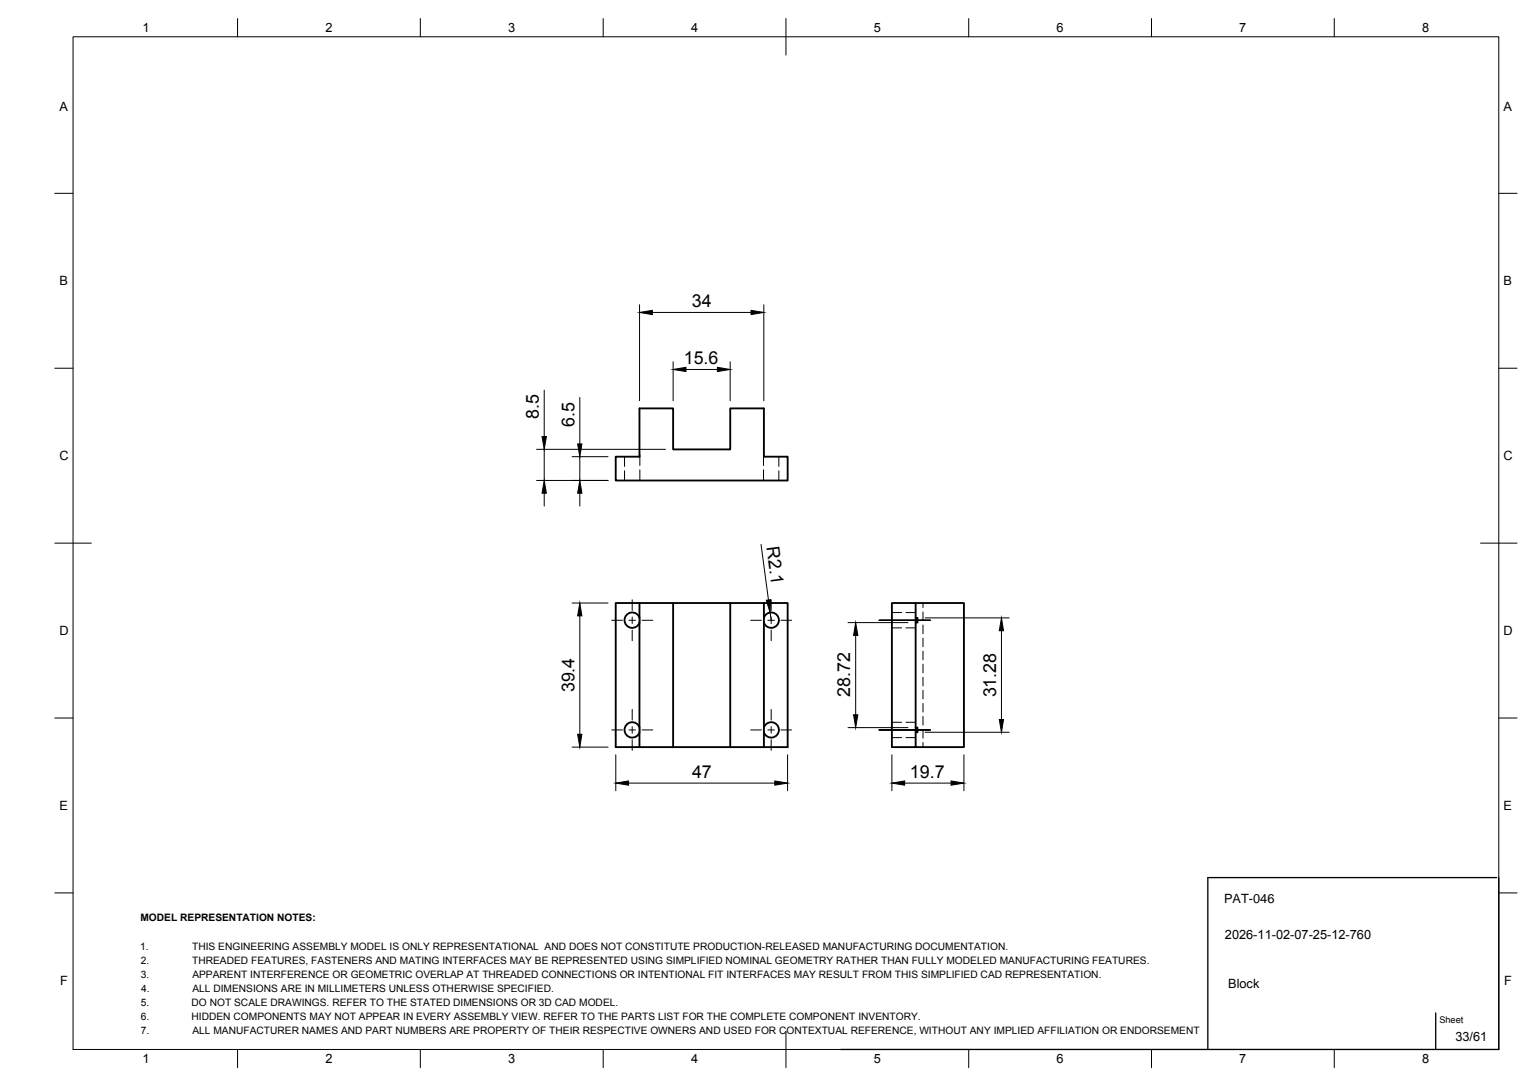
ISO-10303-21;
HEADER;
/* Generated by software containing ST-Developer
 * from STEP Tools, Inc. (www.steptools.com) 
 */

FILE_DESCRIPTION(
/* description */ ('Gear mesh backlash fixture'),
/* implementation_level */ '2;1');

FILE_NAME(
/* name */ 'Block.step',
/* time_stamp */ '2026-10-28T03:26:00-07:00',
/* author */ (''),
/* organization */ (''),
/* preprocessor_version */ 'ST-DEVELOPER v20.2',
/* originating_system */ 'Autodesk Translation Framework v15.17.0.0',
/* authorisation */ '');

FILE_SCHEMA (('AUTOMOTIVE_DESIGN { 1 0 10303 214 3 1 1 }'));
ENDSEC;

DATA;
#10=MECHANICAL_DESIGN_GEOMETRIC_PRESENTATION_REPRESENTATION('',(#1046),#57900);
#939=SHAPE_REPRESENTATION_RELATIONSHIP('SRR','None',#58137,#989);
#989=ADVANCED_BREP_SHAPE_REPRESENTATION('',(#1110),#57870);
#1046=STYLED_ITEM('',(#58444),#1110);
#1110=MANIFOLD_SOLID_BREP('Body1',#13607);
#1276=FACE_BOUND('',#2886,.T.);
#1277=FACE_BOUND('',#2887,.T.);
#1278=FACE_BOUND('',#2888,.T.);
#1279=FACE_BOUND('',#2889,.T.);
#1474=PLANE('',#14803);
#1475=PLANE('',#14809);
#1476=PLANE('',#14815);
#1477=PLANE('',#14821);
#1478=PLANE('',#14827);
#1479=PLANE('',#14828);
#1480=PLANE('',#14829);
#1481=PLANE('',#14830);
#1482=PLANE('',#14831);
#1483=PLANE('',#14832);
#1484=PLANE('',#14833);
#1485=PLANE('',#14834);
#1486=PLANE('',#14835);
#1487=PLANE('',#14836);
#1488=PLANE('',#14837);
#1489=PLANE('',#14838);
#1490=PLANE('',#14839);
#1491=PLANE('',#14840);
#1974=FACE_OUTER_BOUND('',#2872,.T.);
#1975=FACE_OUTER_BOUND('',#2873,.T.);
#1976=FACE_OUTER_BOUND('',#2874,.T.);
#1977=FACE_OUTER_BOUND('',#2875,.T.);
#1978=FACE_OUTER_BOUND('',#2876,.T.);
#1979=FACE_OUTER_BOUND('',#2877,.T.);
#1980=FACE_OUTER_BOUND('',#2878,.T.);
#1981=FACE_OUTER_BOUND('',#2879,.T.);
#1982=FACE_OUTER_BOUND('',#2880,.T.);
#1983=FACE_OUTER_BOUND('',#2881,.T.);
#1984=FACE_OUTER_BOUND('',#2882,.T.);
#1985=FACE_OUTER_BOUND('',#2883,.T.);
#1986=FACE_OUTER_BOUND('',#2884,.T.);
#1987=FACE_OUTER_BOUND('',#2885,.T.);
#1988=FACE_OUTER_BOUND('',#2890,.T.);
#1989=FACE_OUTER_BOUND('',#2891,.T.);
#1990=FACE_OUTER_BOUND('',#2892,.T.);
#1991=FACE_OUTER_BOUND('',#2893,.T.);
#1992=FACE_OUTER_BOUND('',#2894,.T.);
#1993=FACE_OUTER_BOUND('',#2895,.T.);
#1994=FACE_OUTER_BOUND('',#2896,.T.);
#1995=FACE_OUTER_BOUND('',#2897,.T.);
#2872=EDGE_LOOP('',(#10125,#10126));
#2873=EDGE_LOOP('',(#10127,#10128,#10129,#10130,#10131,#10132,#10133,#10134));
#2874=EDGE_LOOP('',(#10135,#10136));
#2875=EDGE_LOOP('',(#10137,#10138,#10139,#10140,#10141,#10142,#10143,#10144));
#2876=EDGE_LOOP('',(#10145,#10146));
#2877=EDGE_LOOP('',(#10147,#10148,#10149,#10150,#10151,#10152,#10153,#10154));
#2878=EDGE_LOOP('',(#10155,#10156));
#2879=EDGE_LOOP('',(#10157,#10158,#10159,#10160,#10161,#10162,#10163,#10164));
#2880=EDGE_LOOP('',(#10165,#10166,#10167,#10168,#10169,#10170,#10171,#10172,
#10173,#10174,#10175,#10176));
#2881=EDGE_LOOP('',(#10177,#10178,#10179,#10180,#10181,#10182,#10183,#10184,
#10185,#10186,#10187,#10188));
#2882=EDGE_LOOP('',(#10189,#10190,#10191,#10192,#10193,#10194,#10195,#10196,
#10197,#10198,#10199,#10200));
#2883=EDGE_LOOP('',(#10201,#10202,#10203,#10204,#10205,#10206,#10207,#10208,
#10209,#10210));
#2884=EDGE_LOOP('',(#10211,#10212,#10213,#10214));
#2885=EDGE_LOOP('',(#10215,#10216,#10217,#10218));
#2886=EDGE_LOOP('',(#10219));
#2887=EDGE_LOOP('',(#10220));
#2888=EDGE_LOOP('',(#10221));
#2889=EDGE_LOOP('',(#10222));
#2890=EDGE_LOOP('',(#10223,#10224,#10225,#10226));
#2891=EDGE_LOOP('',(#10227,#10228,#10229,#10230,#10231,#10232,#10233,#10234,
#10235,#10236));
#2892=EDGE_LOOP('',(#10237,#10238,#10239,#10240));
#2893=EDGE_LOOP('',(#10241,#10242,#10243,#10244));
#2894=EDGE_LOOP('',(#10245,#10246,#10247,#10248));
#2895=EDGE_LOOP('',(#10249,#10250,#10251,#10252));
#2896=EDGE_LOOP('',(#10253,#10254,#10255,#10256));
#2897=EDGE_LOOP('',(#10257,#10258,#10259,#10260,#10261,#10262,#10263,#10264,
#10265,#10266,#10267,#10268));
#3715=LINE('',#21048,#4604);
#3716=LINE('',#21052,#4605);
#3717=LINE('',#21056,#4606);
#3718=LINE('',#21060,#4607);
#3719=LINE('',#21064,#4608);
#3720=LINE('',#21068,#4609);
#3721=LINE('',#21072,#4610);
#3722=LINE('',#21076,#4611);
#3723=LINE('',#21080,#4612);
#3724=LINE('',#21084,#4613);
#3725=LINE('',#21088,#4614);
#3726=LINE('',#21092,#4615);
#3727=LINE('',#21096,#4616);
#3728=LINE('',#21100,#4617);
#3729=LINE('',#21104,#4618);
#3730=LINE('',#21108,#4619);
#3731=LINE('',#21110,#4620);
#3732=LINE('',#21112,#4621);
#3733=LINE('',#21114,#4622);
#3734=LINE('',#21116,#4623);
#3735=LINE('',#21118,#4624);
#3736=LINE('',#21119,#4625);
#3737=LINE('',#21121,#4626);
#3738=LINE('',#21123,#4627);
#3739=LINE('',#21125,#4628);
#3740=LINE('',#21127,#4629);
#3741=LINE('',#21129,#4630);
#3742=LINE('',#21130,#4631);
#3743=LINE('',#21133,#4632);
#3744=LINE('',#21135,#4633);
#3745=LINE('',#21137,#4634);
#3746=LINE('',#21139,#4635);
#3747=LINE('',#21140,#4636);
#3748=LINE('',#21142,#4637);
#3749=LINE('',#21144,#4638);
#3750=LINE('',#21146,#4639);
#3751=LINE('',#21148,#4640);
#3752=LINE('',#21149,#4641);
#3753=LINE('',#21152,#4642);
#3754=LINE('',#21153,#4643);
#3755=LINE('',#21156,#4644);
#3756=LINE('',#21157,#4645);
#3757=LINE('',#21160,#4646);
#3758=LINE('',#21161,#4647);
#3759=LINE('',#21164,#4648);
#3760=LINE('',#21165,#4649);
#3761=LINE('',#21167,#4650);
#3762=LINE('',#21170,#4651);
#3763=LINE('',#21171,#4652);
#3764=LINE('',#21174,#4653);
#3765=LINE('',#21175,#4654);
#3766=LINE('',#21178,#4655);
#3767=LINE('',#21179,#4656);
#3768=LINE('',#21182,#4657);
#3769=LINE('',#21183,#4658);
#3770=LINE('',#21185,#4659);
#4604=VECTOR('',#17100,1.);
#4605=VECTOR('',#17105,1.);
#4606=VECTOR('',#17108,0.21);
#4607=VECTOR('',#17113,1.);
#4608=VECTOR('',#17116,1.);
#4609=VECTOR('',#17121,1.);
#4610=VECTOR('',#17124,0.21);
#4611=VECTOR('',#17129,1.);
#4612=VECTOR('',#17132,1.);
#4613=VECTOR('',#17137,1.);
#4614=VECTOR('',#17140,0.21);
#4615=VECTOR('',#17145,1.);
#4616=VECTOR('',#17148,1.);
#4617=VECTOR('',#17153,1.);
#4618=VECTOR('',#17156,0.21);
#4619=VECTOR('',#17161,1.);
#4620=VECTOR('',#17164,1.);
#4621=VECTOR('',#17165,1.);
#4622=VECTOR('',#17166,1.);
#4623=VECTOR('',#17167,1.);
#4624=VECTOR('',#17168,1.);
#4625=VECTOR('',#17169,1.);
#4626=VECTOR('',#17172,1.);
#4627=VECTOR('',#17173,1.);
#4628=VECTOR('',#17174,1.);
#4629=VECTOR('',#17175,1.);
#4630=VECTOR('',#17176,1.);
#4631=VECTOR('',#17177,1.);
#4632=VECTOR('',#17180,1.);
#4633=VECTOR('',#17181,1.);
#4634=VECTOR('',#17182,1.);
#4635=VECTOR('',#17183,1.);
#4636=VECTOR('',#17184,1.);
#4637=VECTOR('',#17185,1.);
#4638=VECTOR('',#17186,1.);
#4639=VECTOR('',#17187,1.);
#4640=VECTOR('',#17188,1.);
#4641=VECTOR('',#17189,1.);
#4642=VECTOR('',#17192,1.);
#4643=VECTOR('',#17193,1.);
#4644=VECTOR('',#17196,1.);
#4645=VECTOR('',#17197,1.);
#4646=VECTOR('',#17200,1.);
#4647=VECTOR('',#17201,1.);
#4648=VECTOR('',#17204,1.);
#4649=VECTOR('',#17205,1.);
#4650=VECTOR('',#17208,1.);
#4651=VECTOR('',#17211,1.);
#4652=VECTOR('',#17212,1.);
#4653=VECTOR('',#17215,1.);
#4654=VECTOR('',#17216,1.);
#4655=VECTOR('',#17219,1.);
#4656=VECTOR('',#17220,1.);
#4657=VECTOR('',#17223,1.);
#4658=VECTOR('',#17224,1.);
#4659=VECTOR('',#17227,1.);
#5483=CIRCLE('',#14804,0.21);
#5484=CIRCLE('',#14806,0.21);
#5485=CIRCLE('',#14807,0.21);
#5486=CIRCLE('',#14808,0.21);
#5487=CIRCLE('',#14810,0.21);
#5488=CIRCLE('',#14812,0.21);
#5489=CIRCLE('',#14813,0.21);
#5490=CIRCLE('',#14814,0.21);
#5491=CIRCLE('',#14816,0.21);
#5492=CIRCLE('',#14818,0.21);
#5493=CIRCLE('',#14819,0.21);
#5494=CIRCLE('',#14820,0.21);
#5495=CIRCLE('',#14822,0.21);
#5496=CIRCLE('',#14824,0.21);
#5497=CIRCLE('',#14825,0.21);
#5498=CIRCLE('',#14826,0.21);
#6199=VERTEX_POINT('',#21046);
#6200=VERTEX_POINT('',#21047);
#6201=VERTEX_POINT('',#21051);
#6202=VERTEX_POINT('',#21053);
#6203=VERTEX_POINT('',#21055);
#6204=VERTEX_POINT('',#21058);
#6205=VERTEX_POINT('',#21062);
#6206=VERTEX_POINT('',#21063);
#6207=VERTEX_POINT('',#21067);
#6208=VERTEX_POINT('',#21069);
#6209=VERTEX_POINT('',#21071);
#6210=VERTEX_POINT('',#21074);
#6211=VERTEX_POINT('',#21078);
#6212=VERTEX_POINT('',#21079);
#6213=VERTEX_POINT('',#21083);
#6214=VERTEX_POINT('',#21085);
#6215=VERTEX_POINT('',#21087);
#6216=VERTEX_POINT('',#21090);
#6217=VERTEX_POINT('',#21094);
#6218=VERTEX_POINT('',#21095);
#6219=VERTEX_POINT('',#21099);
#6220=VERTEX_POINT('',#21101);
#6221=VERTEX_POINT('',#21103);
#6222=VERTEX_POINT('',#21106);
#6223=VERTEX_POINT('',#21111);
#6224=VERTEX_POINT('',#21113);
#6225=VERTEX_POINT('',#21115);
#6226=VERTEX_POINT('',#21117);
#6227=VERTEX_POINT('',#21122);
#6228=VERTEX_POINT('',#21124);
#6229=VERTEX_POINT('',#21126);
#6230=VERTEX_POINT('',#21128);
#6231=VERTEX_POINT('',#21132);
#6232=VERTEX_POINT('',#21134);
#6233=VERTEX_POINT('',#21136);
#6234=VERTEX_POINT('',#21138);
#6235=VERTEX_POINT('',#21141);
#6236=VERTEX_POINT('',#21143);
#6237=VERTEX_POINT('',#21145);
#6238=VERTEX_POINT('',#21147);
#6239=VERTEX_POINT('',#21151);
#6240=VERTEX_POINT('',#21155);
#6241=VERTEX_POINT('',#21159);
#6242=VERTEX_POINT('',#21163);
#6243=VERTEX_POINT('',#21169);
#6244=VERTEX_POINT('',#21173);
#6245=VERTEX_POINT('',#21177);
#6246=VERTEX_POINT('',#21181);
#7649=EDGE_CURVE('',#6199,#6200,#3715,.T.);
#7650=EDGE_CURVE('',#6199,#6200,#5483,.T.);
#7651=EDGE_CURVE('',#6201,#6199,#3716,.T.);
#7652=EDGE_CURVE('',#6202,#6201,#5484,.T.);
#7653=EDGE_CURVE('',#6202,#6203,#3717,.T.);
#7654=EDGE_CURVE('',#6203,#6203,#5485,.T.);
#7655=EDGE_CURVE('',#6204,#6202,#5486,.T.);
#7656=EDGE_CURVE('',#6200,#6204,#3718,.T.);
#7657=EDGE_CURVE('',#6205,#6206,#3719,.T.);
#7658=EDGE_CURVE('',#6205,#6206,#5487,.T.);
#7659=EDGE_CURVE('',#6207,#6205,#3720,.T.);
#7660=EDGE_CURVE('',#6208,#6207,#5488,.T.);
#7661=EDGE_CURVE('',#6208,#6209,#3721,.T.);
#7662=EDGE_CURVE('',#6209,#6209,#5489,.T.);
#7663=EDGE_CURVE('',#6210,#6208,#5490,.T.);
#7664=EDGE_CURVE('',#6206,#6210,#3722,.T.);
#7665=EDGE_CURVE('',#6211,#6212,#3723,.T.);
#7666=EDGE_CURVE('',#6211,#6212,#5491,.T.);
#7667=EDGE_CURVE('',#6213,#6211,#3724,.T.);
#7668=EDGE_CURVE('',#6214,#6213,#5492,.T.);
#7669=EDGE_CURVE('',#6214,#6215,#3725,.T.);
#7670=EDGE_CURVE('',#6215,#6215,#5493,.T.);
#7671=EDGE_CURVE('',#6216,#6214,#5494,.T.);
#7672=EDGE_CURVE('',#6212,#6216,#3726,.T.);
#7673=EDGE_CURVE('',#6217,#6218,#3727,.T.);
#7674=EDGE_CURVE('',#6217,#6218,#5495,.T.);
#7675=EDGE_CURVE('',#6219,#6217,#3728,.T.);
#7676=EDGE_CURVE('',#6220,#6219,#5496,.T.);
#7677=EDGE_CURVE('',#6220,#6221,#3729,.T.);
#7678=EDGE_CURVE('',#6221,#6221,#5497,.T.);
#7679=EDGE_CURVE('',#6222,#6220,#5498,.T.);
#7680=EDGE_CURVE('',#6218,#6222,#3730,.T.);
#7681=EDGE_CURVE('',#6204,#6213,#3731,.T.);
#7682=EDGE_CURVE('',#6216,#6223,#3732,.T.);
#7683=EDGE_CURVE('',#6224,#6223,#3733,.T.);
#7684=EDGE_CURVE('',#6224,#6225,#3734,.T.);
#7685=EDGE_CURVE('',#6226,#6225,#3735,.T.);
#7686=EDGE_CURVE('',#6226,#6201,#3736,.T.);
#7687=EDGE_CURVE('',#6210,#6219,#3737,.T.);
#7688=EDGE_CURVE('',#6222,#6227,#3738,.T.);
#7689=EDGE_CURVE('',#6228,#6227,#3739,.T.);
#7690=EDGE_CURVE('',#6229,#6228,#3740,.T.);
#7691=EDGE_CURVE('',#6230,#6229,#3741,.T.);
#7692=EDGE_CURVE('',#6230,#6207,#3742,.T.);
#7693=EDGE_CURVE('',#6223,#6231,#3743,.T.);
#7694=EDGE_CURVE('',#6231,#6232,#3744,.T.);
#7695=EDGE_CURVE('',#6232,#6233,#3745,.T.);
#7696=EDGE_CURVE('',#6233,#6234,#3746,.T.);
#7697=EDGE_CURVE('',#6234,#6230,#3747,.T.);
#7698=EDGE_CURVE('',#6229,#6235,#3748,.T.);
#7699=EDGE_CURVE('',#6235,#6236,#3749,.T.);
#7700=EDGE_CURVE('',#6236,#6237,#3750,.T.);
#7701=EDGE_CURVE('',#6237,#6238,#3751,.T.);
#7702=EDGE_CURVE('',#6238,#6224,#3752,.T.);
#7703=EDGE_CURVE('',#6239,#6226,#3753,.T.);
#7704=EDGE_CURVE('',#6231,#6239,#3754,.T.);
#7705=EDGE_CURVE('',#6240,#6239,#3755,.T.);
#7706=EDGE_CURVE('',#6232,#6240,#3756,.T.);
#7707=EDGE_CURVE('',#6241,#6240,#3757,.T.);
#7708=EDGE_CURVE('',#6233,#6241,#3758,.T.);
#7709=EDGE_CURVE('',#6242,#6241,#3759,.T.);
#7710=EDGE_CURVE('',#6234,#6242,#3760,.T.);
#7711=EDGE_CURVE('',#6227,#6242,#3761,.T.);
#7712=EDGE_CURVE('',#6243,#6228,#3762,.T.);
#7713=EDGE_CURVE('',#6235,#6243,#3763,.T.);
#7714=EDGE_CURVE('',#6244,#6243,#3764,.T.);
#7715=EDGE_CURVE('',#6236,#6244,#3765,.T.);
#7716=EDGE_CURVE('',#6245,#6244,#3766,.T.);
#7717=EDGE_CURVE('',#6237,#6245,#3767,.T.);
#7718=EDGE_CURVE('',#6246,#6245,#3768,.T.);
#7719=EDGE_CURVE('',#6238,#6246,#3769,.T.);
#7720=EDGE_CURVE('',#6225,#6246,#3770,.T.);
#10125=ORIENTED_EDGE('',*,*,#7649,.F.);
#10126=ORIENTED_EDGE('',*,*,#7650,.T.);
#10127=ORIENTED_EDGE('',*,*,#7651,.F.);
#10128=ORIENTED_EDGE('',*,*,#7652,.F.);
#10129=ORIENTED_EDGE('',*,*,#7653,.T.);
#10130=ORIENTED_EDGE('',*,*,#7654,.F.);
#10131=ORIENTED_EDGE('',*,*,#7653,.F.);
#10132=ORIENTED_EDGE('',*,*,#7655,.F.);
#10133=ORIENTED_EDGE('',*,*,#7656,.F.);
#10134=ORIENTED_EDGE('',*,*,#7650,.F.);
#10135=ORIENTED_EDGE('',*,*,#7657,.F.);
#10136=ORIENTED_EDGE('',*,*,#7658,.T.);
#10137=ORIENTED_EDGE('',*,*,#7659,.F.);
#10138=ORIENTED_EDGE('',*,*,#7660,.F.);
#10139=ORIENTED_EDGE('',*,*,#7661,.T.);
#10140=ORIENTED_EDGE('',*,*,#7662,.F.);
#10141=ORIENTED_EDGE('',*,*,#7661,.F.);
#10142=ORIENTED_EDGE('',*,*,#7663,.F.);
#10143=ORIENTED_EDGE('',*,*,#7664,.F.);
#10144=ORIENTED_EDGE('',*,*,#7658,.F.);
#10145=ORIENTED_EDGE('',*,*,#7665,.F.);
#10146=ORIENTED_EDGE('',*,*,#7666,.T.);
#10147=ORIENTED_EDGE('',*,*,#7667,.F.);
#10148=ORIENTED_EDGE('',*,*,#7668,.F.);
#10149=ORIENTED_EDGE('',*,*,#7669,.T.);
#10150=ORIENTED_EDGE('',*,*,#7670,.F.);
#10151=ORIENTED_EDGE('',*,*,#7669,.F.);
#10152=ORIENTED_EDGE('',*,*,#7671,.F.);
#10153=ORIENTED_EDGE('',*,*,#7672,.F.);
#10154=ORIENTED_EDGE('',*,*,#7666,.F.);
#10155=ORIENTED_EDGE('',*,*,#7673,.F.);
#10156=ORIENTED_EDGE('',*,*,#7674,.T.);
#10157=ORIENTED_EDGE('',*,*,#7675,.F.);
#10158=ORIENTED_EDGE('',*,*,#7676,.F.);
#10159=ORIENTED_EDGE('',*,*,#7677,.T.);
#10160=ORIENTED_EDGE('',*,*,#7678,.F.);
#10161=ORIENTED_EDGE('',*,*,#7677,.F.);
#10162=ORIENTED_EDGE('',*,*,#7679,.F.);
#10163=ORIENTED_EDGE('',*,*,#7680,.F.);
#10164=ORIENTED_EDGE('',*,*,#7674,.F.);
#10165=ORIENTED_EDGE('',*,*,#7651,.T.);
#10166=ORIENTED_EDGE('',*,*,#7649,.T.);
#10167=ORIENTED_EDGE('',*,*,#7656,.T.);
#10168=ORIENTED_EDGE('',*,*,#7681,.T.);
#10169=ORIENTED_EDGE('',*,*,#7667,.T.);
#10170=ORIENTED_EDGE('',*,*,#7665,.T.);
#10171=ORIENTED_EDGE('',*,*,#7672,.T.);
#10172=ORIENTED_EDGE('',*,*,#7682,.T.);
#10173=ORIENTED_EDGE('',*,*,#7683,.F.);
#10174=ORIENTED_EDGE('',*,*,#7684,.T.);
#10175=ORIENTED_EDGE('',*,*,#7685,.F.);
#10176=ORIENTED_EDGE('',*,*,#7686,.T.);
#10177=ORIENTED_EDGE('',*,*,#7659,.T.);
#10178=ORIENTED_EDGE('',*,*,#7657,.T.);
#10179=ORIENTED_EDGE('',*,*,#7664,.T.);
#10180=ORIENTED_EDGE('',*,*,#7687,.T.);
#10181=ORIENTED_EDGE('',*,*,#7675,.T.);
#10182=ORIENTED_EDGE('',*,*,#7673,.T.);
#10183=ORIENTED_EDGE('',*,*,#7680,.T.);
#10184=ORIENTED_EDGE('',*,*,#7688,.T.);
#10185=ORIENTED_EDGE('',*,*,#7689,.F.);
#10186=ORIENTED_EDGE('',*,*,#7690,.F.);
#10187=ORIENTED_EDGE('',*,*,#7691,.F.);
#10188=ORIENTED_EDGE('',*,*,#7692,.T.);
#10189=ORIENTED_EDGE('',*,*,#7683,.T.);
#10190=ORIENTED_EDGE('',*,*,#7693,.T.);
#10191=ORIENTED_EDGE('',*,*,#7694,.T.);
#10192=ORIENTED_EDGE('',*,*,#7695,.T.);
#10193=ORIENTED_EDGE('',*,*,#7696,.T.);
#10194=ORIENTED_EDGE('',*,*,#7697,.T.);
#10195=ORIENTED_EDGE('',*,*,#7691,.T.);
#10196=ORIENTED_EDGE('',*,*,#7698,.T.);
#10197=ORIENTED_EDGE('',*,*,#7699,.T.);
#10198=ORIENTED_EDGE('',*,*,#7700,.T.);
#10199=ORIENTED_EDGE('',*,*,#7701,.T.);
#10200=ORIENTED_EDGE('',*,*,#7702,.T.);
#10201=ORIENTED_EDGE('',*,*,#7655,.T.);
#10202=ORIENTED_EDGE('',*,*,#7652,.T.);
#10203=ORIENTED_EDGE('',*,*,#7686,.F.);
#10204=ORIENTED_EDGE('',*,*,#7703,.F.);
#10205=ORIENTED_EDGE('',*,*,#7704,.F.);
#10206=ORIENTED_EDGE('',*,*,#7693,.F.);
#10207=ORIENTED_EDGE('',*,*,#7682,.F.);
#10208=ORIENTED_EDGE('',*,*,#7671,.T.);
#10209=ORIENTED_EDGE('',*,*,#7668,.T.);
#10210=ORIENTED_EDGE('',*,*,#7681,.F.);
#10211=ORIENTED_EDGE('',*,*,#7704,.T.);
#10212=ORIENTED_EDGE('',*,*,#7705,.F.);
#10213=ORIENTED_EDGE('',*,*,#7706,.F.);
#10214=ORIENTED_EDGE('',*,*,#7694,.F.);
#10215=ORIENTED_EDGE('',*,*,#7706,.T.);
#10216=ORIENTED_EDGE('',*,*,#7707,.F.);
#10217=ORIENTED_EDGE('',*,*,#7708,.F.);
#10218=ORIENTED_EDGE('',*,*,#7695,.F.);
#10219=ORIENTED_EDGE('',*,*,#7654,.T.);
#10220=ORIENTED_EDGE('',*,*,#7662,.T.);
#10221=ORIENTED_EDGE('',*,*,#7670,.T.);
#10222=ORIENTED_EDGE('',*,*,#7678,.T.);
#10223=ORIENTED_EDGE('',*,*,#7708,.T.);
#10224=ORIENTED_EDGE('',*,*,#7709,.F.);
#10225=ORIENTED_EDGE('',*,*,#7710,.F.);
#10226=ORIENTED_EDGE('',*,*,#7696,.F.);
#10227=ORIENTED_EDGE('',*,*,#7663,.T.);
#10228=ORIENTED_EDGE('',*,*,#7660,.T.);
#10229=ORIENTED_EDGE('',*,*,#7692,.F.);
#10230=ORIENTED_EDGE('',*,*,#7697,.F.);
#10231=ORIENTED_EDGE('',*,*,#7710,.T.);
#10232=ORIENTED_EDGE('',*,*,#7711,.F.);
#10233=ORIENTED_EDGE('',*,*,#7688,.F.);
#10234=ORIENTED_EDGE('',*,*,#7679,.T.);
#10235=ORIENTED_EDGE('',*,*,#7676,.T.);
#10236=ORIENTED_EDGE('',*,*,#7687,.F.);
#10237=ORIENTED_EDGE('',*,*,#7690,.T.);
#10238=ORIENTED_EDGE('',*,*,#7712,.F.);
#10239=ORIENTED_EDGE('',*,*,#7713,.F.);
#10240=ORIENTED_EDGE('',*,*,#7698,.F.);
#10241=ORIENTED_EDGE('',*,*,#7713,.T.);
#10242=ORIENTED_EDGE('',*,*,#7714,.F.);
#10243=ORIENTED_EDGE('',*,*,#7715,.F.);
#10244=ORIENTED_EDGE('',*,*,#7699,.F.);
#10245=ORIENTED_EDGE('',*,*,#7715,.T.);
#10246=ORIENTED_EDGE('',*,*,#7716,.F.);
#10247=ORIENTED_EDGE('',*,*,#7717,.F.);
#10248=ORIENTED_EDGE('',*,*,#7700,.F.);
#10249=ORIENTED_EDGE('',*,*,#7717,.T.);
#10250=ORIENTED_EDGE('',*,*,#7718,.F.);
#10251=ORIENTED_EDGE('',*,*,#7719,.F.);
#10252=ORIENTED_EDGE('',*,*,#7701,.F.);
#10253=ORIENTED_EDGE('',*,*,#7719,.T.);
#10254=ORIENTED_EDGE('',*,*,#7720,.F.);
#10255=ORIENTED_EDGE('',*,*,#7684,.F.);
#10256=ORIENTED_EDGE('',*,*,#7702,.F.);
#10257=ORIENTED_EDGE('',*,*,#7685,.T.);
#10258=ORIENTED_EDGE('',*,*,#7720,.T.);
#10259=ORIENTED_EDGE('',*,*,#7718,.T.);
#10260=ORIENTED_EDGE('',*,*,#7716,.T.);
#10261=ORIENTED_EDGE('',*,*,#7714,.T.);
#10262=ORIENTED_EDGE('',*,*,#7712,.T.);
#10263=ORIENTED_EDGE('',*,*,#7689,.T.);
#10264=ORIENTED_EDGE('',*,*,#7711,.T.);
#10265=ORIENTED_EDGE('',*,*,#7709,.T.);
#10266=ORIENTED_EDGE('',*,*,#7707,.T.);
#10267=ORIENTED_EDGE('',*,*,#7705,.T.);
#10268=ORIENTED_EDGE('',*,*,#7703,.T.);
#12697=CYLINDRICAL_SURFACE('',#14805,0.21);
#12698=CYLINDRICAL_SURFACE('',#14811,0.21);
#12699=CYLINDRICAL_SURFACE('',#14817,0.21);
#12700=CYLINDRICAL_SURFACE('',#14823,0.21);
#13091=ADVANCED_FACE('',(#1974),#1474,.T.);
#13092=ADVANCED_FACE('',(#1975),#12697,.F.);
#13093=ADVANCED_FACE('',(#1976),#1475,.T.);
#13094=ADVANCED_FACE('',(#1977),#12698,.F.);
#13095=ADVANCED_FACE('',(#1978),#1476,.T.);
#13096=ADVANCED_FACE('',(#1979),#12699,.F.);
#13097=ADVANCED_FACE('',(#1980),#1477,.T.);
#13098=ADVANCED_FACE('',(#1981),#12700,.F.);
#13099=ADVANCED_FACE('',(#1982),#1478,.T.);
#13100=ADVANCED_FACE('',(#1983),#1479,.T.);
#13101=ADVANCED_FACE('',(#1984),#1480,.T.);
#13102=ADVANCED_FACE('',(#1985),#1481,.T.);
#13103=ADVANCED_FACE('',(#1986),#1482,.T.);
#13104=ADVANCED_FACE('',(#1987,#1276,#1277,#1278,#1279),#1483,.T.);
#13105=ADVANCED_FACE('',(#1988),#1484,.T.);
#13106=ADVANCED_FACE('',(#1989),#1485,.T.);
#13107=ADVANCED_FACE('',(#1990),#1486,.T.);
#13108=ADVANCED_FACE('',(#1991),#1487,.T.);
#13109=ADVANCED_FACE('',(#1992),#1488,.T.);
#13110=ADVANCED_FACE('',(#1993),#1489,.T.);
#13111=ADVANCED_FACE('',(#1994),#1490,.T.);
#13112=ADVANCED_FACE('',(#1995),#1491,.T.);
#13607=CLOSED_SHELL('',(#13091,#13092,#13093,#13094,#13095,#13096,#13097,
#13098,#13099,#13100,#13101,#13102,#13103,#13104,#13105,#13106,#13107,#13108,
#13109,#13110,#13111,#13112));
#14802=AXIS2_PLACEMENT_3D('',#21044,#17096,#17097);
#14803=AXIS2_PLACEMENT_3D('',#21045,#17098,#17099);
#14804=AXIS2_PLACEMENT_3D('',#21049,#17101,#17102);
#14805=AXIS2_PLACEMENT_3D('',#21050,#17103,#17104);
#14806=AXIS2_PLACEMENT_3D('',#21054,#17106,#17107);
#14807=AXIS2_PLACEMENT_3D('',#21057,#17109,#17110);
#14808=AXIS2_PLACEMENT_3D('',#21059,#17111,#17112);
#14809=AXIS2_PLACEMENT_3D('',#21061,#17114,#17115);
#14810=AXIS2_PLACEMENT_3D('',#21065,#17117,#17118);
#14811=AXIS2_PLACEMENT_3D('',#21066,#17119,#17120);
#14812=AXIS2_PLACEMENT_3D('',#21070,#17122,#17123);
#14813=AXIS2_PLACEMENT_3D('',#21073,#17125,#17126);
#14814=AXIS2_PLACEMENT_3D('',#21075,#17127,#17128);
#14815=AXIS2_PLACEMENT_3D('',#21077,#17130,#17131);
#14816=AXIS2_PLACEMENT_3D('',#21081,#17133,#17134);
#14817=AXIS2_PLACEMENT_3D('',#21082,#17135,#17136);
#14818=AXIS2_PLACEMENT_3D('',#21086,#17138,#17139);
#14819=AXIS2_PLACEMENT_3D('',#21089,#17141,#17142);
#14820=AXIS2_PLACEMENT_3D('',#21091,#17143,#17144);
#14821=AXIS2_PLACEMENT_3D('',#21093,#17146,#17147);
#14822=AXIS2_PLACEMENT_3D('',#21097,#17149,#17150);
#14823=AXIS2_PLACEMENT_3D('',#21098,#17151,#17152);
#14824=AXIS2_PLACEMENT_3D('',#21102,#17154,#17155);
#14825=AXIS2_PLACEMENT_3D('',#21105,#17157,#17158);
#14826=AXIS2_PLACEMENT_3D('',#21107,#17159,#17160);
#14827=AXIS2_PLACEMENT_3D('',#21109,#17162,#17163);
#14828=AXIS2_PLACEMENT_3D('',#21120,#17170,#17171);
#14829=AXIS2_PLACEMENT_3D('',#21131,#17178,#17179);
#14830=AXIS2_PLACEMENT_3D('',#21150,#17190,#17191);
#14831=AXIS2_PLACEMENT_3D('',#21154,#17194,#17195);
#14832=AXIS2_PLACEMENT_3D('',#21158,#17198,#17199);
#14833=AXIS2_PLACEMENT_3D('',#21162,#17202,#17203);
#14834=AXIS2_PLACEMENT_3D('',#21166,#17206,#17207);
#14835=AXIS2_PLACEMENT_3D('',#21168,#17209,#17210);
#14836=AXIS2_PLACEMENT_3D('',#21172,#17213,#17214);
#14837=AXIS2_PLACEMENT_3D('',#21176,#17217,#17218);
#14838=AXIS2_PLACEMENT_3D('',#21180,#17221,#17222);
#14839=AXIS2_PLACEMENT_3D('',#21184,#17225,#17226);
#14840=AXIS2_PLACEMENT_3D('',#21186,#17228,#17229);
#17096=DIRECTION('axis',(0.,0.,1.));
#17097=DIRECTION('refdir',(1.,0.,0.));
#17098=DIRECTION('center_axis',(0.,0.,1.));
#17099=DIRECTION('ref_axis',(1.,0.,0.));
#17100=DIRECTION('',(-1.,0.,0.));
#17101=DIRECTION('center_axis',(0.,0.,1.));
#17102=DIRECTION('ref_axis',(1.,0.,0.));
#17103=DIRECTION('center_axis',(0.,0.,1.));
#17104=DIRECTION('ref_axis',(1.,0.,0.));
#17105=DIRECTION('',(0.,0.,-1.));
#17106=DIRECTION('center_axis',(0.,0.,1.));
#17107=DIRECTION('ref_axis',(1.,0.,0.));
#17108=DIRECTION('',(0.,0.,1.));
#17109=DIRECTION('center_axis',(0.,0.,-1.));
#17110=DIRECTION('ref_axis',(1.,0.,0.));
#17111=DIRECTION('center_axis',(0.,0.,1.));
#17112=DIRECTION('ref_axis',(1.,0.,0.));
#17113=DIRECTION('',(0.,0.,1.));
#17114=DIRECTION('center_axis',(0.,0.,1.));
#17115=DIRECTION('ref_axis',(1.,0.,0.));
#17116=DIRECTION('',(1.,0.,0.));
#17117=DIRECTION('center_axis',(0.,0.,1.));
#17118=DIRECTION('ref_axis',(1.,0.,0.));
#17119=DIRECTION('center_axis',(0.,0.,1.));
#17120=DIRECTION('ref_axis',(1.,0.,0.));
#17121=DIRECTION('',(0.,0.,-1.));
#17122=DIRECTION('center_axis',(0.,0.,1.));
#17123=DIRECTION('ref_axis',(1.,0.,0.));
#17124=DIRECTION('',(0.,0.,1.));
#17125=DIRECTION('center_axis',(0.,0.,-1.));
#17126=DIRECTION('ref_axis',(1.,0.,0.));
#17127=DIRECTION('center_axis',(0.,0.,1.));
#17128=DIRECTION('ref_axis',(1.,0.,0.));
#17129=DIRECTION('',(0.,0.,1.));
#17130=DIRECTION('center_axis',(0.,0.,1.));
#17131=DIRECTION('ref_axis',(1.,0.,0.));
#17132=DIRECTION('',(-1.,0.,0.));
#17133=DIRECTION('center_axis',(0.,0.,1.));
#17134=DIRECTION('ref_axis',(1.,0.,0.));
#17135=DIRECTION('center_axis',(0.,0.,1.));
#17136=DIRECTION('ref_axis',(1.,0.,0.));
#17137=DIRECTION('',(0.,0.,-1.));
#17138=DIRECTION('center_axis',(0.,0.,1.));
#17139=DIRECTION('ref_axis',(1.,0.,0.));
#17140=DIRECTION('',(0.,0.,1.));
#17141=DIRECTION('center_axis',(0.,0.,-1.));
#17142=DIRECTION('ref_axis',(1.,0.,0.));
#17143=DIRECTION('center_axis',(0.,0.,1.));
#17144=DIRECTION('ref_axis',(1.,0.,0.));
#17145=DIRECTION('',(0.,0.,1.));
#17146=DIRECTION('center_axis',(0.,0.,1.));
#17147=DIRECTION('ref_axis',(1.,0.,0.));
#17148=DIRECTION('',(1.,0.,0.));
#17149=DIRECTION('center_axis',(0.,0.,1.));
#17150=DIRECTION('ref_axis',(1.,0.,0.));
#17151=DIRECTION('center_axis',(0.,0.,1.));
#17152=DIRECTION('ref_axis',(1.,0.,0.));
#17153=DIRECTION('',(0.,0.,-1.));
#17154=DIRECTION('center_axis',(0.,0.,1.));
#17155=DIRECTION('ref_axis',(1.,0.,0.));
#17156=DIRECTION('',(0.,0.,1.));
#17157=DIRECTION('center_axis',(0.,0.,-1.));
#17158=DIRECTION('ref_axis',(1.,0.,0.));
#17159=DIRECTION('center_axis',(0.,0.,1.));
#17160=DIRECTION('ref_axis',(1.,0.,0.));
#17161=DIRECTION('',(0.,0.,1.));
#17162=DIRECTION('center_axis',(0.,-1.,0.));
#17163=DIRECTION('ref_axis',(0.,0.,-1.));
#17164=DIRECTION('',(-1.,0.,0.));
#17165=DIRECTION('',(-1.,0.,0.));
#17166=DIRECTION('',(0.,0.,1.));
#17167=DIRECTION('',(1.,0.,0.));
#17168=DIRECTION('',(0.,0.,-1.));
#17169=DIRECTION('',(-1.,0.,0.));
#17170=DIRECTION('center_axis',(0.,1.,0.));
#17171=DIRECTION('ref_axis',(0.,0.,1.));
#17172=DIRECTION('',(1.,0.,0.));
#17173=DIRECTION('',(1.,0.,0.));
#17174=DIRECTION('',(0.,0.,1.));
#17175=DIRECTION('',(1.,0.,0.));
#17176=DIRECTION('',(0.,0.,-1.));
#17177=DIRECTION('',(1.,0.,0.));
#17178=DIRECTION('center_axis',(-1.,0.,0.));
#17179=DIRECTION('ref_axis',(0.,0.,1.));
#17180=DIRECTION('',(0.,-1.,0.));
#17181=DIRECTION('',(0.,0.,1.));
#17182=DIRECTION('',(0.,1.,0.));
#17183=DIRECTION('',(0.,0.,-1.));
#17184=DIRECTION('',(0.,-1.,0.));
#17185=DIRECTION('',(0.,-1.,0.));
#17186=DIRECTION('',(0.,0.,1.));
#17187=DIRECTION('',(0.,-1.,0.));
#17188=DIRECTION('',(0.,0.,-1.));
#17189=DIRECTION('',(0.,-1.,0.));
#17190=DIRECTION('center_axis',(0.,0.,-1.));
#17191=DIRECTION('ref_axis',(0.,1.,0.));
#17192=DIRECTION('',(0.,1.,0.));
#17193=DIRECTION('',(1.,0.,0.));
#17194=DIRECTION('center_axis',(0.,-1.,0.));
#17195=DIRECTION('ref_axis',(0.,0.,-1.));
#17196=DIRECTION('',(0.,0.,-1.));
#17197=DIRECTION('',(1.,0.,0.));
#17198=DIRECTION('center_axis',(0.,0.,1.));
#17199=DIRECTION('ref_axis',(0.,-1.,0.));
#17200=DIRECTION('',(0.,-1.,0.));
#17201=DIRECTION('',(1.,0.,0.));
#17202=DIRECTION('center_axis',(0.,1.,0.));
#17203=DIRECTION('ref_axis',(0.,0.,1.));
#17204=DIRECTION('',(0.,0.,1.));
#17205=DIRECTION('',(1.,0.,0.));
#17206=DIRECTION('center_axis',(0.,0.,-1.));
#17207=DIRECTION('ref_axis',(0.,1.,0.));
#17208=DIRECTION('',(0.,1.,0.));
#17209=DIRECTION('center_axis',(0.,0.,-1.));
#17210=DIRECTION('ref_axis',(0.,1.,0.));
#17211=DIRECTION('',(0.,1.,0.));
#17212=DIRECTION('',(1.,0.,0.));
#17213=DIRECTION('center_axis',(0.,-1.,0.));
#17214=DIRECTION('ref_axis',(0.,0.,-1.));
#17215=DIRECTION('',(0.,0.,-1.));
#17216=DIRECTION('',(1.,0.,0.));
#17217=DIRECTION('center_axis',(0.,0.,-1.));
#17218=DIRECTION('ref_axis',(0.,1.,0.));
#17219=DIRECTION('',(0.,1.,0.));
#17220=DIRECTION('',(1.,0.,0.));
#17221=DIRECTION('center_axis',(0.,1.,0.));
#17222=DIRECTION('ref_axis',(0.,0.,1.));
#17223=DIRECTION('',(0.,0.,1.));
#17224=DIRECTION('',(1.,0.,0.));
#17225=DIRECTION('center_axis',(0.,0.,-1.));
#17226=DIRECTION('ref_axis',(0.,1.,0.));
#17227=DIRECTION('',(0.,1.,0.));
#17228=DIRECTION('center_axis',(1.,0.,0.));
#17229=DIRECTION('ref_axis',(0.,0.,-1.));
#21044=CARTESIAN_POINT('',(0.,0.,0.));
#21045=CARTESIAN_POINT('Origin',(1.5,-1.9,1.7));
#21046=CARTESIAN_POINT('',(1.56403124237433,-1.7,1.7));
#21047=CARTESIAN_POINT('',(1.43596875762567,-1.7,1.7));
#21048=CARTESIAN_POINT('',(0.75,-1.7,1.7));
#21049=CARTESIAN_POINT('Origin',(1.5,-1.9,1.7));
#21050=CARTESIAN_POINT('Origin',(1.5,-1.9,1.7));
#21051=CARTESIAN_POINT('',(1.56403124237433,-1.7,1.75));
#21052=CARTESIAN_POINT('',(1.56403124237433,-1.7,1.7));
#21053=CARTESIAN_POINT('',(1.29,-1.9,1.75));
#21054=CARTESIAN_POINT('Origin',(1.5,-1.9,1.75));
#21055=CARTESIAN_POINT('',(1.29,-1.9,2.4));
#21056=CARTESIAN_POINT('',(1.29,-1.9,1.7));
#21057=CARTESIAN_POINT('Origin',(1.5,-1.9,2.4));
#21058=CARTESIAN_POINT('',(1.43596875762567,-1.7,1.75));
#21059=CARTESIAN_POINT('Origin',(1.5,-1.9,1.75));
#21060=CARTESIAN_POINT('',(1.43596875762567,-1.7,1.7));
#21061=CARTESIAN_POINT('Origin',(-1.5,1.9,1.7));
#21062=CARTESIAN_POINT('',(-1.56403124237433,1.7,1.7));
#21063=CARTESIAN_POINT('',(-1.43596875762567,1.7,1.7));
#21064=CARTESIAN_POINT('',(-0.75,1.7,1.7));
#21065=CARTESIAN_POINT('Origin',(-1.5,1.9,1.7));
#21066=CARTESIAN_POINT('Origin',(-1.5,1.9,1.7));
#21067=CARTESIAN_POINT('',(-1.56403124237433,1.7,1.75));
#21068=CARTESIAN_POINT('',(-1.56403124237433,1.7,1.7));
#21069=CARTESIAN_POINT('',(-1.71,1.9,1.75));
#21070=CARTESIAN_POINT('Origin',(-1.5,1.9,1.75));
#21071=CARTESIAN_POINT('',(-1.71,1.9,2.4));
#21072=CARTESIAN_POINT('',(-1.71,1.9,1.7));
#21073=CARTESIAN_POINT('Origin',(-1.5,1.9,2.4));
#21074=CARTESIAN_POINT('',(-1.43596875762567,1.7,1.75));
#21075=CARTESIAN_POINT('Origin',(-1.5,1.9,1.75));
#21076=CARTESIAN_POINT('',(-1.43596875762567,1.7,1.7));
#21077=CARTESIAN_POINT('Origin',(-1.5,-1.9,1.7));
#21078=CARTESIAN_POINT('',(-1.43596875762567,-1.7,1.7));
#21079=CARTESIAN_POINT('',(-1.56403124237433,-1.7,1.7));
#21080=CARTESIAN_POINT('',(-0.75,-1.7,1.7));
#21081=CARTESIAN_POINT('Origin',(-1.5,-1.9,1.7));
#21082=CARTESIAN_POINT('Origin',(-1.5,-1.9,1.7));
#21083=CARTESIAN_POINT('',(-1.43596875762567,-1.7,1.75));
#21084=CARTESIAN_POINT('',(-1.43596875762567,-1.7,1.7));
#21085=CARTESIAN_POINT('',(-1.71,-1.9,1.75));
#21086=CARTESIAN_POINT('Origin',(-1.5,-1.9,1.75));
#21087=CARTESIAN_POINT('',(-1.71,-1.9,2.4));
#21088=CARTESIAN_POINT('',(-1.71,-1.9,1.7));
#21089=CARTESIAN_POINT('Origin',(-1.5,-1.9,2.4));
#21090=CARTESIAN_POINT('',(-1.56403124237433,-1.7,1.75));
#21091=CARTESIAN_POINT('Origin',(-1.5,-1.9,1.75));
#21092=CARTESIAN_POINT('',(-1.56403124237433,-1.7,1.7));
#21093=CARTESIAN_POINT('Origin',(1.5,1.9,1.7));
#21094=CARTESIAN_POINT('',(1.43596875762567,1.7,1.7));
#21095=CARTESIAN_POINT('',(1.56403124237433,1.7,1.7));
#21096=CARTESIAN_POINT('',(0.75,1.7,1.7));
#21097=CARTESIAN_POINT('Origin',(1.5,1.9,1.7));
#21098=CARTESIAN_POINT('Origin',(1.5,1.9,1.7));
#21099=CARTESIAN_POINT('',(1.43596875762567,1.7,1.75));
#21100=CARTESIAN_POINT('',(1.43596875762567,1.7,1.7));
#21101=CARTESIAN_POINT('',(1.29,1.9,1.75));
#21102=CARTESIAN_POINT('Origin',(1.5,1.9,1.75));
#21103=CARTESIAN_POINT('',(1.29,1.9,2.4));
#21104=CARTESIAN_POINT('',(1.29,1.9,1.7));
#21105=CARTESIAN_POINT('Origin',(1.5,1.9,2.4));
#21106=CARTESIAN_POINT('',(1.56403124237433,1.7,1.75));
#21107=CARTESIAN_POINT('Origin',(1.5,1.9,1.75));
#21108=CARTESIAN_POINT('',(1.56403124237433,1.7,1.7));
#21109=CARTESIAN_POINT('Origin',(0.,-1.7,1.75));
#21110=CARTESIAN_POINT('',(0.,-1.7,1.75));
#21111=CARTESIAN_POINT('',(-1.97,-1.7,1.75));
#21112=CARTESIAN_POINT('',(0.,-1.7,1.75));
#21113=CARTESIAN_POINT('',(-1.97,-1.7,0.43));
#21114=CARTESIAN_POINT('',(-1.97,-1.7,1.75));
#21115=CARTESIAN_POINT('',(1.97,-1.7,0.43));
#21116=CARTESIAN_POINT('',(0.,-1.7,0.43));
#21117=CARTESIAN_POINT('',(1.97,-1.7,1.75));
#21118=CARTESIAN_POINT('',(1.97,-1.7,1.75));
#21119=CARTESIAN_POINT('',(0.,-1.7,1.75));
#21120=CARTESIAN_POINT('Origin',(0.,1.7,0.43));
#21121=CARTESIAN_POINT('',(0.,1.7,1.75));
#21122=CARTESIAN_POINT('',(1.97,1.7,1.75));
#21123=CARTESIAN_POINT('',(0.,1.7,1.75));
#21124=CARTESIAN_POINT('',(1.97,1.7,0.43));
#21125=CARTESIAN_POINT('',(1.97,1.7,0.43));
#21126=CARTESIAN_POINT('',(-1.97,1.7,0.43));
#21127=CARTESIAN_POINT('',(0.,1.7,0.43));
#21128=CARTESIAN_POINT('',(-1.97,1.7,1.75));
#21129=CARTESIAN_POINT('',(-1.97,1.7,0.43));
#21130=CARTESIAN_POINT('',(0.,1.7,1.75));
#21131=CARTESIAN_POINT('Origin',(-1.97,0.,1.415));
#21132=CARTESIAN_POINT('',(-1.97,-2.35,1.75));
#21133=CARTESIAN_POINT('',(-1.97,-2.35,1.75));
#21134=CARTESIAN_POINT('',(-1.97,-2.35,2.4));
#21135=CARTESIAN_POINT('',(-1.97,-2.35,2.4));
#21136=CARTESIAN_POINT('',(-1.97,2.35,2.4));
#21137=CARTESIAN_POINT('',(-1.97,2.35,2.4));
#21138=CARTESIAN_POINT('',(-1.97,2.35,1.75));
#21139=CARTESIAN_POINT('',(-1.97,2.35,1.75));
#21140=CARTESIAN_POINT('',(-1.97,1.7,1.75));
#21141=CARTESIAN_POINT('',(-1.97,0.78,0.43));
#21142=CARTESIAN_POINT('',(-1.97,0.78,0.43));
#21143=CARTESIAN_POINT('',(-1.97,0.78,1.55));
#21144=CARTESIAN_POINT('',(-1.97,0.78,1.55));
#21145=CARTESIAN_POINT('',(-1.97,-0.78,1.55));
#21146=CARTESIAN_POINT('',(-1.97,-0.78,1.55));
#21147=CARTESIAN_POINT('',(-1.97,-0.78,0.43));
#21148=CARTESIAN_POINT('',(-1.97,-0.78,0.43));
#21149=CARTESIAN_POINT('',(-1.97,-1.7,0.43));
#21150=CARTESIAN_POINT('Origin',(0.,-2.35,1.75));
#21151=CARTESIAN_POINT('',(1.97,-2.35,1.75));
#21152=CARTESIAN_POINT('',(1.97,-2.35,1.75));
#21153=CARTESIAN_POINT('',(0.,-2.35,1.75));
#21154=CARTESIAN_POINT('Origin',(0.,-2.35,2.4));
#21155=CARTESIAN_POINT('',(1.97,-2.35,2.4));
#21156=CARTESIAN_POINT('',(1.97,-2.35,2.4));
#21157=CARTESIAN_POINT('',(0.,-2.35,2.4));
#21158=CARTESIAN_POINT('Origin',(0.,2.35,2.4));
#21159=CARTESIAN_POINT('',(1.97,2.35,2.4));
#21160=CARTESIAN_POINT('',(1.97,2.35,2.4));
#21161=CARTESIAN_POINT('',(0.,2.35,2.4));
#21162=CARTESIAN_POINT('Origin',(0.,2.35,1.75));
#21163=CARTESIAN_POINT('',(1.97,2.35,1.75));
#21164=CARTESIAN_POINT('',(1.97,2.35,1.75));
#21165=CARTESIAN_POINT('',(0.,2.35,1.75));
#21166=CARTESIAN_POINT('Origin',(0.,1.7,1.75));
#21167=CARTESIAN_POINT('',(1.97,1.7,1.75));
#21168=CARTESIAN_POINT('Origin',(0.,0.78,0.43));
#21169=CARTESIAN_POINT('',(1.97,0.78,0.43));
#21170=CARTESIAN_POINT('',(1.97,0.78,0.43));
#21171=CARTESIAN_POINT('',(0.,0.78,0.43));
#21172=CARTESIAN_POINT('Origin',(0.,0.78,1.55));
#21173=CARTESIAN_POINT('',(1.97,0.78,1.55));
#21174=CARTESIAN_POINT('',(1.97,0.78,1.55));
#21175=CARTESIAN_POINT('',(0.,0.78,1.55));
#21176=CARTESIAN_POINT('Origin',(0.,-0.78,1.55));
#21177=CARTESIAN_POINT('',(1.97,-0.78,1.55));
#21178=CARTESIAN_POINT('',(1.97,-0.78,1.55));
#21179=CARTESIAN_POINT('',(0.,-0.78,1.55));
#21180=CARTESIAN_POINT('Origin',(0.,-0.78,0.43));
#21181=CARTESIAN_POINT('',(1.97,-0.78,0.43));
#21182=CARTESIAN_POINT('',(1.97,-0.78,0.43));
#21183=CARTESIAN_POINT('',(0.,-0.78,0.43));
#21184=CARTESIAN_POINT('Origin',(0.,-1.7,0.43));
#21185=CARTESIAN_POINT('',(1.97,-1.7,0.43));
#21186=CARTESIAN_POINT('Origin',(1.97,0.,1.415));
#57811=UNCERTAINTY_MEASURE_WITH_UNIT(LENGTH_MEASURE(0.001),#57901,
'DISTANCE_ACCURACY_VALUE',
'Maximum model space distance between geometric entities at asserted c
onnectivities');
#57841=UNCERTAINTY_MEASURE_WITH_UNIT(LENGTH_MEASURE(0.001),#57901,
'DISTANCE_ACCURACY_VALUE',
'Maximum model space distance between geometric entities at asserted c
onnectivities');
#57870=(
GEOMETRIC_REPRESENTATION_CONTEXT(3)
GLOBAL_UNCERTAINTY_ASSIGNED_CONTEXT((#57811))
GLOBAL_UNIT_ASSIGNED_CONTEXT((#57901,#57903,#57904))
REPRESENTATION_CONTEXT('','3D')
);
#57900=(
GEOMETRIC_REPRESENTATION_CONTEXT(3)
GLOBAL_UNCERTAINTY_ASSIGNED_CONTEXT((#57841))
GLOBAL_UNIT_ASSIGNED_CONTEXT((#57901,#57903,#57904))
REPRESENTATION_CONTEXT('','3D')
);
#57901=(
LENGTH_UNIT()
NAMED_UNIT(*)
SI_UNIT(.CENTI.,.METRE.)
);
#57903=(
NAMED_UNIT(*)
PLANE_ANGLE_UNIT()
SI_UNIT($,.RADIAN.)
);
#57904=(
NAMED_UNIT(*)
SI_UNIT($,.STERADIAN.)
SOLID_ANGLE_UNIT()
);
#57933=SHAPE_DEFINITION_REPRESENTATION(#57996,#58137);
#57996=PRODUCT_DEFINITION_SHAPE('',$,#58196);
#58137=SHAPE_REPRESENTATION('',(#14802),#57870);
#58167=PRODUCT_DEFINITION_CONTEXT('part definition',#58343,'design');
#58196=PRODUCT_DEFINITION('Block','Block',#58254,#58167);
#58254=PRODUCT_DEFINITION_FORMATION('',$,#58373);
#58343=APPLICATION_CONTEXT(
'Core Data for Automotive Mechanical Design Process');
#58344=PRODUCT_CONTEXT('part definition',#58343,'mechanical');
#58373=PRODUCT('Block','Block','Block',(#58344));
#58438=COLOUR_RGB('Dark Blue',0.08,0.2,0.34);
#58439=FILL_AREA_STYLE_COLOUR('',#58438);
#58440=FILL_AREA_STYLE('',(#58439));
#58441=SURFACE_STYLE_FILL_AREA(#58440);
#58442=SURFACE_SIDE_STYLE('',(#58441));
#58443=SURFACE_STYLE_USAGE(.BOTH.,#58442);
#58444=PRESENTATION_STYLE_ASSIGNMENT((#58443));
ENDSEC;
END-ISO-10303-21;
